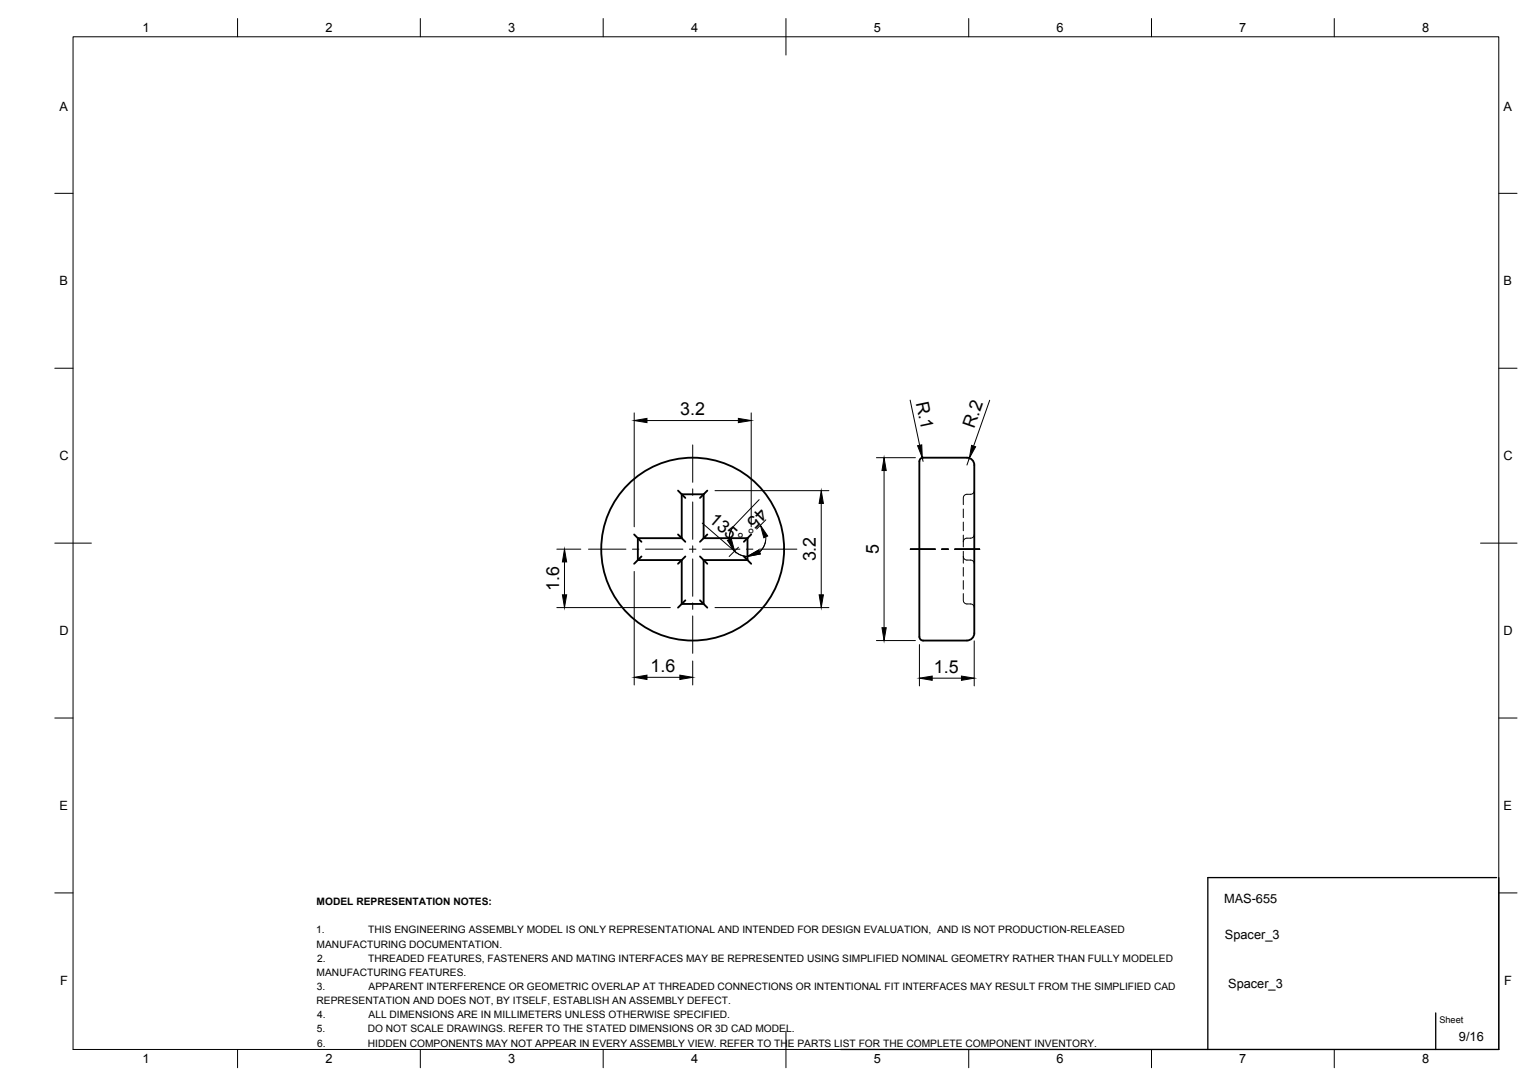
ISO-10303-21;
HEADER;
FILE_DESCRIPTION((''),'2;1');
FILE_NAME('Spacer_3.step','2026-10-09T11:34:15-07:00',(''),(''),'','','');
FILE_SCHEMA (('AUTOMOTIVE_DESIGN { 1 0 10303 214 3 1 1 }'));
ENDSEC;
DATA;
#10=MECHANICAL_DESIGN_GEOMETRIC_PRESENTATION_REPRESENTATION('',(#641),#117170);
#365=ELLIPSE('',#52371,0.141421356237294,0.1) ;
#366=ELLIPSE('',#52372,0.141421356237322,0.1) ;
#367=ELLIPSE('',#52374,0.141421356237325,0.1) ;
#368=ELLIPSE('',#52376,0.141421356237297,0.1) ;
#369=ELLIPSE('',#52378,0.141421356237322,0.1) ;
#370=ELLIPSE('',#52380,0.141421356237297,0.1) ;
#371=ELLIPSE('',#52382,0.141421356237322,0.1) ;
#372=ELLIPSE('',#52384,0.141421356237294,0.1) ;
#373=ELLIPSE('',#52386,0.141421356237325,0.1) ;
#374=ELLIPSE('',#52388,0.141421356237297,0.1) ;
#375=ELLIPSE('',#52390,0.141421356237322,0.1) ;
#376=ELLIPSE('',#52392,0.141421356237297,0.1) ;
#377=ELLIPSE('',#52411,0.141421356237297,0.1) ;
#378=ELLIPSE('',#52412,0.141421356237322,0.1) ;
#379=ELLIPSE('',#52414,0.141421356237322,0.1) ;
#380=ELLIPSE('',#52416,0.141421356237297,0.1) ;
#381=ELLIPSE('',#52418,0.141421356237322,0.1) ;
#382=ELLIPSE('',#52420,0.141421356237297,0.1) ;
#383=ELLIPSE('',#52422,0.141421356237297,0.1) ;
#384=ELLIPSE('',#52423,0.141421356237297,0.1) ;
#385=ELLIPSE('',#52425,0.141421356237322,0.1) ;
#386=ELLIPSE('',#52428,0.141421356237297,0.1) ;
#387=ELLIPSE('',#52430,0.141421356237322,0.1) ;
#388=ELLIPSE('',#52432,0.141421356237297,0.1) ;
#599=SHAPE_REPRESENTATION_RELATIONSHIP('SRR','None',#117254,#620) ;
#620=ADVANCED_BREP_SHAPE_REPRESENTATION('',(#662),#117162) ;
#641=STYLED_ITEM('',(#117355),#662) ;
#662=MANIFOLD_SOLID_BREP('Body1',#49070) ;
#736=FACE_BOUND('',#15495,.T.) ;
#2537=PLANE('',#52394) ;
#2538=PLANE('',#52395) ;
#2539=PLANE('',#52396) ;
#2540=PLANE('',#52397) ;
#2541=PLANE('',#52398) ;
#2542=PLANE('',#52399) ;
#2543=PLANE('',#52400) ;
#2544=PLANE('',#52409) ;
#2545=PLANE('',#52434) ;
#2546=PLANE('',#52435) ;
#2547=PLANE('',#52436) ;
#2548=PLANE('',#52437) ;
#2549=PLANE('',#52441) ;
#2550=PLANE('',#52442) ;
#2551=PLANE('',#52443) ;
#4488=LINE('',#88586,#7702) ;
#4489=LINE('',#88590,#7703) ;
#4490=LINE('',#88594,#7704) ;
#4491=LINE('',#88597,#7705) ;
#4492=LINE('',#88600,#7706) ;
#4493=LINE('',#88603,#7707) ;
#4494=LINE('',#88606,#7708) ;
#4495=LINE('',#88609,#7709) ;
#4496=LINE('',#88612,#7710) ;
#4497=LINE('',#88615,#7711) ;
#4498=LINE('',#88618,#7712) ;
#4499=LINE('',#88620,#7713) ;
#4500=LINE('',#88624,#7714) ;
#4501=LINE('',#88626,#7715) ;
#4502=LINE('',#88630,#7716) ;
#4503=LINE('',#88632,#7717) ;
#4504=LINE('',#88636,#7718) ;
#4505=LINE('',#88638,#7719) ;
#4506=LINE('',#88642,#7720) ;
#4507=LINE('',#88644,#7721) ;
#4508=LINE('',#88648,#7722) ;
#4509=LINE('',#88650,#7723) ;
#4510=LINE('',#88653,#7724) ;
#4511=LINE('',#88654,#7725) ;
#4512=LINE('',#88657,#7726) ;
#4513=LINE('',#88659,#7727) ;
#4514=LINE('',#88660,#7728) ;
#4515=LINE('',#88663,#7729) ;
#4516=LINE('',#88664,#7730) ;
#4517=LINE('',#88667,#7731) ;
#4518=LINE('',#88668,#7732) ;
#4519=LINE('',#88671,#7733) ;
#4520=LINE('',#88672,#7734) ;
#4521=LINE('',#88675,#7735) ;
#4522=LINE('',#88676,#7736) ;
#4523=LINE('',#88679,#7737) ;
#4524=LINE('',#88680,#7738) ;
#4525=LINE('',#88692,#7739) ;
#4526=LINE('',#88700,#7740) ;
#4527=LINE('',#88705,#7741) ;
#4528=LINE('',#88709,#7742) ;
#4529=LINE('',#88713,#7743) ;
#4530=LINE('',#88717,#7744) ;
#4531=LINE('',#88720,#7745) ;
#4532=LINE('',#88724,#7746) ;
#4533=LINE('',#88728,#7747) ;
#4534=LINE('',#88732,#7748) ;
#4535=LINE('',#88734,#7749) ;
#4536=LINE('',#88737,#7750) ;
#4537=LINE('',#88738,#7751) ;
#4538=LINE('',#88741,#7752) ;
#4539=LINE('',#88743,#7753) ;
#4540=LINE('',#88746,#7754) ;
#4541=LINE('',#88748,#7755) ;
#4542=LINE('',#88752,#7756) ;
#4543=LINE('',#88755,#7757) ;
#4544=LINE('',#88757,#7758) ;
#4545=LINE('',#88759,#7759) ;
#4546=LINE('',#88761,#7760) ;
#4547=LINE('',#88768,#7761) ;
#4548=LINE('',#88770,#7762) ;
#7702=VECTOR('',#62675,10.) ;
#7703=VECTOR('',#62678,10.) ;
#7704=VECTOR('',#62683,10.) ;
#7705=VECTOR('',#62686,10.) ;
#7706=VECTOR('',#62689,10.) ;
#7707=VECTOR('',#62692,10.) ;
#7708=VECTOR('',#62695,10.) ;
#7709=VECTOR('',#62698,10.) ;
#7710=VECTOR('',#62701,10.) ;
#7711=VECTOR('',#62704,10.) ;
#7712=VECTOR('',#62707,10.) ;
#7713=VECTOR('',#62708,10.) ;
#7714=VECTOR('',#62713,10.) ;
#7715=VECTOR('',#62714,10.) ;
#7716=VECTOR('',#62719,10.) ;
#7717=VECTOR('',#62720,10.) ;
#7718=VECTOR('',#62725,10.) ;
#7719=VECTOR('',#62726,10.) ;
#7720=VECTOR('',#62731,10.) ;
#7721=VECTOR('',#62732,10.) ;
#7722=VECTOR('',#62737,10.) ;
#7723=VECTOR('',#62738,10.) ;
#7724=VECTOR('',#62743,10.) ;
#7725=VECTOR('',#62744,10.) ;
#7726=VECTOR('',#62747,10.) ;
#7727=VECTOR('',#62748,10.) ;
#7728=VECTOR('',#62749,10.) ;
#7729=VECTOR('',#62752,10.) ;
#7730=VECTOR('',#62753,10.) ;
#7731=VECTOR('',#62756,10.) ;
#7732=VECTOR('',#62757,10.) ;
#7733=VECTOR('',#62760,10.) ;
#7734=VECTOR('',#62761,10.) ;
#7735=VECTOR('',#62764,10.) ;
#7736=VECTOR('',#62765,10.) ;
#7737=VECTOR('',#62768,10.) ;
#7738=VECTOR('',#62769,10.) ;
#7739=VECTOR('',#62784,2.5) ;
#7740=VECTOR('',#62793,10.) ;
#7741=VECTOR('',#62800,10.) ;
#7742=VECTOR('',#62805,10.) ;
#7743=VECTOR('',#62810,10.) ;
#7744=VECTOR('',#62815,10.) ;
#7745=VECTOR('',#62818,10.) ;
#7746=VECTOR('',#62821,10.) ;
#7747=VECTOR('',#62824,10.) ;
#7748=VECTOR('',#62829,10.) ;
#7749=VECTOR('',#62830,10.) ;
#7750=VECTOR('',#62835,10.) ;
#7751=VECTOR('',#62836,10.) ;
#7752=VECTOR('',#62839,10.) ;
#7753=VECTOR('',#62840,10.) ;
#7754=VECTOR('',#62845,10.) ;
#7755=VECTOR('',#62846,10.) ;
#7756=VECTOR('',#62851,10.) ;
#7757=VECTOR('',#62856,10.) ;
#7758=VECTOR('',#62859,10.) ;
#7759=VECTOR('',#62862,10.) ;
#7760=VECTOR('',#62865,10.) ;
#7761=VECTOR('',#62876,10.) ;
#7762=VECTOR('',#62879,10.) ;
#10090=CYLINDRICAL_SURFACE('',#52370,0.1) ;
#10091=CYLINDRICAL_SURFACE('',#52373,0.1) ;
#10092=CYLINDRICAL_SURFACE('',#52375,0.1) ;
#10093=CYLINDRICAL_SURFACE('',#52377,0.1) ;
#10094=CYLINDRICAL_SURFACE('',#52379,0.1) ;
#10095=CYLINDRICAL_SURFACE('',#52381,0.1) ;
#10096=CYLINDRICAL_SURFACE('',#52383,0.1) ;
#10097=CYLINDRICAL_SURFACE('',#52385,0.1) ;
#10098=CYLINDRICAL_SURFACE('',#52387,0.1) ;
#10099=CYLINDRICAL_SURFACE('',#52389,0.1) ;
#10100=CYLINDRICAL_SURFACE('',#52391,0.1) ;
#10101=CYLINDRICAL_SURFACE('',#52393,0.1) ;
#10102=CYLINDRICAL_SURFACE('',#52406,2.5) ;
#10103=CYLINDRICAL_SURFACE('',#52410,0.1) ;
#10104=CYLINDRICAL_SURFACE('',#52413,0.1) ;
#10105=CYLINDRICAL_SURFACE('',#52415,0.1) ;
#10106=CYLINDRICAL_SURFACE('',#52417,0.1) ;
#10107=CYLINDRICAL_SURFACE('',#52419,0.1) ;
#10108=CYLINDRICAL_SURFACE('',#52421,0.1) ;
#10109=CYLINDRICAL_SURFACE('',#52424,0.1) ;
#10110=CYLINDRICAL_SURFACE('',#52426,0.1) ;
#10111=CYLINDRICAL_SURFACE('',#52427,0.1) ;
#10112=CYLINDRICAL_SURFACE('',#52429,0.1) ;
#10113=CYLINDRICAL_SURFACE('',#52431,0.1) ;
#10114=CYLINDRICAL_SURFACE('',#52433,0.1) ;
#12299=FACE_OUTER_BOUND('',#15457,.T.) ;
#12300=FACE_OUTER_BOUND('',#15458,.T.) ;
#12301=FACE_OUTER_BOUND('',#15459,.T.) ;
#12302=FACE_OUTER_BOUND('',#15460,.T.) ;
#12303=FACE_OUTER_BOUND('',#15461,.T.) ;
#12304=FACE_OUTER_BOUND('',#15462,.T.) ;
#12305=FACE_OUTER_BOUND('',#15463,.T.) ;
#12306=FACE_OUTER_BOUND('',#15464,.T.) ;
#12307=FACE_OUTER_BOUND('',#15465,.T.) ;
#12308=FACE_OUTER_BOUND('',#15466,.T.) ;
#12309=FACE_OUTER_BOUND('',#15467,.T.) ;
#12310=FACE_OUTER_BOUND('',#15468,.T.) ;
#12311=FACE_OUTER_BOUND('',#15469,.T.) ;
#12312=FACE_OUTER_BOUND('',#15470,.T.) ;
#12313=FACE_OUTER_BOUND('',#15471,.T.) ;
#12314=FACE_OUTER_BOUND('',#15472,.T.) ;
#12315=FACE_OUTER_BOUND('',#15473,.T.) ;
#12316=FACE_OUTER_BOUND('',#15474,.T.) ;
#12317=FACE_OUTER_BOUND('',#15475,.T.) ;
#12318=FACE_OUTER_BOUND('',#15476,.T.) ;
#12319=FACE_OUTER_BOUND('',#15477,.T.) ;
#12320=FACE_OUTER_BOUND('',#15478,.T.) ;
#12321=FACE_OUTER_BOUND('',#15479,.T.) ;
#12322=FACE_OUTER_BOUND('',#15480,.T.) ;
#12323=FACE_OUTER_BOUND('',#15481,.T.) ;
#12324=FACE_OUTER_BOUND('',#15482,.T.) ;
#12325=FACE_OUTER_BOUND('',#15483,.T.) ;
#12326=FACE_OUTER_BOUND('',#15484,.T.) ;
#12327=FACE_OUTER_BOUND('',#15485,.T.) ;
#12328=FACE_OUTER_BOUND('',#15486,.T.) ;
#12329=FACE_OUTER_BOUND('',#15487,.T.) ;
#12330=FACE_OUTER_BOUND('',#15488,.T.) ;
#12331=FACE_OUTER_BOUND('',#15489,.T.) ;
#12332=FACE_OUTER_BOUND('',#15490,.T.) ;
#12333=FACE_OUTER_BOUND('',#15491,.T.) ;
#12334=FACE_OUTER_BOUND('',#15492,.T.) ;
#12335=FACE_OUTER_BOUND('',#15493,.T.) ;
#12336=FACE_OUTER_BOUND('',#15494,.T.) ;
#12337=FACE_OUTER_BOUND('',#15496,.T.) ;
#12338=FACE_OUTER_BOUND('',#15497,.T.) ;
#12339=FACE_OUTER_BOUND('',#15498,.T.) ;
#12340=FACE_OUTER_BOUND('',#15499,.T.) ;
#15457=EDGE_LOOP('',(#38114,#38115,#38116,#38117)) ;
#15458=EDGE_LOOP('',(#38118,#38119,#38120,#38121)) ;
#15459=EDGE_LOOP('',(#38122,#38123,#38124,#38125)) ;
#15460=EDGE_LOOP('',(#38126,#38127,#38128,#38129)) ;
#15461=EDGE_LOOP('',(#38130,#38131,#38132,#38133)) ;
#15462=EDGE_LOOP('',(#38134,#38135,#38136,#38137)) ;
#15463=EDGE_LOOP('',(#38138,#38139,#38140,#38141)) ;
#15464=EDGE_LOOP('',(#38142,#38143,#38144,#38145)) ;
#15465=EDGE_LOOP('',(#38146,#38147,#38148,#38149)) ;
#15466=EDGE_LOOP('',(#38150,#38151,#38152,#38153)) ;
#15467=EDGE_LOOP('',(#38154,#38155,#38156,#38157)) ;
#15468=EDGE_LOOP('',(#38158,#38159,#38160,#38161)) ;
#15469=EDGE_LOOP('',(#38162,#38163,#38164,#38165)) ;
#15470=EDGE_LOOP('',(#38166,#38167,#38168,#38169)) ;
#15471=EDGE_LOOP('',(#38170,#38171,#38172,#38173)) ;
#15472=EDGE_LOOP('',(#38174,#38175,#38176,#38177)) ;
#15473=EDGE_LOOP('',(#38178,#38179,#38180,#38181)) ;
#15474=EDGE_LOOP('',(#38182,#38183,#38184,#38185)) ;
#15475=EDGE_LOOP('',(#38186,#38187,#38188,#38189,#38190,#38191,#38192,#38193,
#38194,#38195,#38196,#38197)) ;
#15476=EDGE_LOOP('',(#38198,#38199,#38200,#38201,#38202)) ;
#15477=EDGE_LOOP('',(#38203,#38204,#38205,#38206,#38207,#38208)) ;
#15478=EDGE_LOOP('',(#38209)) ;
#15479=EDGE_LOOP('',(#38210,#38211,#38212,#38213)) ;
#15480=EDGE_LOOP('',(#38214,#38215,#38216,#38217)) ;
#15481=EDGE_LOOP('',(#38218,#38219,#38220,#38221)) ;
#15482=EDGE_LOOP('',(#38222,#38223,#38224,#38225)) ;
#15483=EDGE_LOOP('',(#38226,#38227,#38228,#38229)) ;
#15484=EDGE_LOOP('',(#38230,#38231,#38232,#38233)) ;
#15485=EDGE_LOOP('',(#38234,#38235,#38236,#38237)) ;
#15486=EDGE_LOOP('',(#38238,#38239,#38240,#38241)) ;
#15487=EDGE_LOOP('',(#38242,#38243,#38244,#38245)) ;
#15488=EDGE_LOOP('',(#38246,#38247,#38248,#38249)) ;
#15489=EDGE_LOOP('',(#38250,#38251,#38252,#38253)) ;
#15490=EDGE_LOOP('',(#38254,#38255,#38256,#38257)) ;
#15491=EDGE_LOOP('',(#38258,#38259,#38260,#38261)) ;
#15492=EDGE_LOOP('',(#38262,#38263,#38264,#38265)) ;
#15493=EDGE_LOOP('',(#38266,#38267,#38268,#38269)) ;
#15494=EDGE_LOOP('',(#38270)) ;
#15495=EDGE_LOOP('',(#38271,#38272,#38273,#38274,#38275,#38276,#38277,#38278,
#38279,#38280,#38281,#38282)) ;
#15496=EDGE_LOOP('',(#38283,#38284,#38285,#38286,#38287)) ;
#15497=EDGE_LOOP('',(#38288,#38289,#38290,#38291)) ;
#15498=EDGE_LOOP('',(#38292,#38293,#38294,#38295)) ;
#15499=EDGE_LOOP('',(#38296,#38297,#38298,#38299)) ;
#18501=CIRCLE('',#52402,2.4) ;
#18502=CIRCLE('',#52403,0.1) ;
#18503=CIRCLE('',#52404,2.5) ;
#18504=CIRCLE('',#52405,2.5) ;
#18505=CIRCLE('',#52407,2.5) ;
#18506=CIRCLE('',#52408,2.5) ;
#18507=CIRCLE('',#52438,2.3) ;
#18508=CIRCLE('',#52440,0.2) ;
#21615=VERTEX_POINT('',#88584) ;
#21616=VERTEX_POINT('',#88585) ;
#21617=VERTEX_POINT('',#88587) ;
#21618=VERTEX_POINT('',#88589) ;
#21619=VERTEX_POINT('',#88593) ;
#21620=VERTEX_POINT('',#88595) ;
#21621=VERTEX_POINT('',#88599) ;
#21622=VERTEX_POINT('',#88601) ;
#21623=VERTEX_POINT('',#88605) ;
#21624=VERTEX_POINT('',#88607) ;
#21625=VERTEX_POINT('',#88611) ;
#21626=VERTEX_POINT('',#88613) ;
#21627=VERTEX_POINT('',#88617) ;
#21628=VERTEX_POINT('',#88619) ;
#21629=VERTEX_POINT('',#88623) ;
#21630=VERTEX_POINT('',#88625) ;
#21631=VERTEX_POINT('',#88629) ;
#21632=VERTEX_POINT('',#88631) ;
#21633=VERTEX_POINT('',#88635) ;
#21634=VERTEX_POINT('',#88637) ;
#21635=VERTEX_POINT('',#88641) ;
#21636=VERTEX_POINT('',#88643) ;
#21637=VERTEX_POINT('',#88647) ;
#21638=VERTEX_POINT('',#88649) ;
#21639=VERTEX_POINT('',#88656) ;
#21640=VERTEX_POINT('',#88658) ;
#21641=VERTEX_POINT('',#88662) ;
#21642=VERTEX_POINT('',#88666) ;
#21643=VERTEX_POINT('',#88670) ;
#21644=VERTEX_POINT('',#88674) ;
#21645=VERTEX_POINT('',#88678) ;
#21646=VERTEX_POINT('',#88683) ;
#21647=VERTEX_POINT('',#88685) ;
#21648=VERTEX_POINT('',#88687) ;
#21649=VERTEX_POINT('',#88691) ;
#21650=VERTEX_POINT('',#88693) ;
#21651=VERTEX_POINT('',#88698) ;
#21652=VERTEX_POINT('',#88699) ;
#21653=VERTEX_POINT('',#88704) ;
#21654=VERTEX_POINT('',#88708) ;
#21655=VERTEX_POINT('',#88712) ;
#21656=VERTEX_POINT('',#88716) ;
#21657=VERTEX_POINT('',#88718) ;
#21658=VERTEX_POINT('',#88722) ;
#21659=VERTEX_POINT('',#88723) ;
#21660=VERTEX_POINT('',#88725) ;
#21661=VERTEX_POINT('',#88727) ;
#21662=VERTEX_POINT('',#88731) ;
#21663=VERTEX_POINT('',#88733) ;
#21664=VERTEX_POINT('',#88740) ;
#21665=VERTEX_POINT('',#88742) ;
#21666=VERTEX_POINT('',#88747) ;
#21667=VERTEX_POINT('',#88751) ;
#21668=VERTEX_POINT('',#88763) ;
#27335=EDGE_CURVE('',#21615,#21616,#4488,.T.) ;
#27336=EDGE_CURVE('',#21616,#21617,#365,.T.) ;
#27337=EDGE_CURVE('',#21617,#21618,#4489,.T.) ;
#27338=EDGE_CURVE('',#21615,#21618,#366,.T.) ;
#27339=EDGE_CURVE('',#21616,#21619,#4490,.T.) ;
#27340=EDGE_CURVE('',#21619,#21620,#367,.T.) ;
#27341=EDGE_CURVE('',#21620,#21617,#4491,.T.) ;
#27342=EDGE_CURVE('',#21619,#21621,#4492,.T.) ;
#27343=EDGE_CURVE('',#21621,#21622,#368,.T.) ;
#27344=EDGE_CURVE('',#21622,#21620,#4493,.T.) ;
#27345=EDGE_CURVE('',#21621,#21623,#4494,.T.) ;
#27346=EDGE_CURVE('',#21623,#21624,#369,.T.) ;
#27347=EDGE_CURVE('',#21624,#21622,#4495,.T.) ;
#27348=EDGE_CURVE('',#21623,#21625,#4496,.T.) ;
#27349=EDGE_CURVE('',#21625,#21626,#370,.T.) ;
#27350=EDGE_CURVE('',#21626,#21624,#4497,.T.) ;
#27351=EDGE_CURVE('',#21627,#21626,#4498,.T.) ;
#27352=EDGE_CURVE('',#21625,#21628,#4499,.T.) ;
#27353=EDGE_CURVE('',#21628,#21627,#371,.T.) ;
#27354=EDGE_CURVE('',#21629,#21627,#4500,.T.) ;
#27355=EDGE_CURVE('',#21628,#21630,#4501,.T.) ;
#27356=EDGE_CURVE('',#21630,#21629,#372,.T.) ;
#27357=EDGE_CURVE('',#21631,#21629,#4502,.T.) ;
#27358=EDGE_CURVE('',#21630,#21632,#4503,.T.) ;
#27359=EDGE_CURVE('',#21632,#21631,#373,.T.) ;
#27360=EDGE_CURVE('',#21633,#21631,#4504,.T.) ;
#27361=EDGE_CURVE('',#21632,#21634,#4505,.T.) ;
#27362=EDGE_CURVE('',#21634,#21633,#374,.T.) ;
#27363=EDGE_CURVE('',#21635,#21633,#4506,.T.) ;
#27364=EDGE_CURVE('',#21634,#21636,#4507,.T.) ;
#27365=EDGE_CURVE('',#21636,#21635,#375,.T.) ;
#27366=EDGE_CURVE('',#21637,#21635,#4508,.T.) ;
#27367=EDGE_CURVE('',#21636,#21638,#4509,.T.) ;
#27368=EDGE_CURVE('',#21638,#21637,#376,.T.) ;
#27369=EDGE_CURVE('',#21618,#21637,#4510,.T.) ;
#27370=EDGE_CURVE('',#21638,#21615,#4511,.T.) ;
#27371=EDGE_CURVE('',#21639,#21631,#4512,.T.) ;
#27372=EDGE_CURVE('',#21640,#21639,#4513,.T.) ;
#27373=EDGE_CURVE('',#21640,#21629,#4514,.T.) ;
#27374=EDGE_CURVE('',#21641,#21633,#4515,.T.) ;
#27375=EDGE_CURVE('',#21639,#21641,#4516,.T.) ;
#27376=EDGE_CURVE('',#21642,#21635,#4517,.T.) ;
#27377=EDGE_CURVE('',#21641,#21642,#4518,.T.) ;
#27378=EDGE_CURVE('',#21643,#21637,#4519,.T.) ;
#27379=EDGE_CURVE('',#21642,#21643,#4520,.T.) ;
#27380=EDGE_CURVE('',#21644,#21618,#4521,.T.) ;
#27381=EDGE_CURVE('',#21643,#21644,#4522,.T.) ;
#27382=EDGE_CURVE('',#21645,#21617,#4523,.T.) ;
#27383=EDGE_CURVE('',#21644,#21645,#4524,.T.) ;
#27384=EDGE_CURVE('',#21646,#21646,#18501,.T.) ;
#27385=EDGE_CURVE('',#21646,#21647,#18502,.T.) ;
#27386=EDGE_CURVE('',#21647,#21648,#18503,.T.) ;
#27387=EDGE_CURVE('',#21648,#21647,#18504,.T.) ;
#27388=EDGE_CURVE('',#21648,#21649,#4525,.T.) ;
#27389=EDGE_CURVE('',#21650,#21649,#18505,.T.) ;
#27390=EDGE_CURVE('',#21649,#21650,#18506,.T.) ;
#27391=EDGE_CURVE('',#21651,#21652,#4526,.T.) ;
#27392=EDGE_CURVE('',#21652,#21642,#377,.T.) ;
#27393=EDGE_CURVE('',#21651,#21643,#378,.T.) ;
#27394=EDGE_CURVE('',#21652,#21653,#4527,.T.) ;
#27395=EDGE_CURVE('',#21653,#21641,#379,.T.) ;
#27396=EDGE_CURVE('',#21653,#21654,#4528,.T.) ;
#27397=EDGE_CURVE('',#21654,#21639,#380,.T.) ;
#27398=EDGE_CURVE('',#21654,#21655,#4529,.T.) ;
#27399=EDGE_CURVE('',#21655,#21640,#381,.T.) ;
#27400=EDGE_CURVE('',#21655,#21656,#4530,.T.) ;
#27401=EDGE_CURVE('',#21656,#21657,#382,.T.) ;
#27402=EDGE_CURVE('',#21657,#21640,#4531,.T.) ;
#27403=EDGE_CURVE('',#21658,#21659,#4532,.T.) ;
#27404=EDGE_CURVE('',#21659,#21660,#383,.T.) ;
#27405=EDGE_CURVE('',#21660,#21661,#4533,.T.) ;
#27406=EDGE_CURVE('',#21661,#21658,#384,.T.) ;
#27407=EDGE_CURVE('',#21662,#21660,#4534,.T.) ;
#27408=EDGE_CURVE('',#21659,#21663,#4535,.T.) ;
#27409=EDGE_CURVE('',#21663,#21662,#385,.T.) ;
#27410=EDGE_CURVE('',#21656,#21658,#4536,.T.) ;
#27411=EDGE_CURVE('',#21661,#21657,#4537,.T.) ;
#27412=EDGE_CURVE('',#21664,#21662,#4538,.T.) ;
#27413=EDGE_CURVE('',#21663,#21665,#4539,.T.) ;
#27414=EDGE_CURVE('',#21665,#21664,#386,.T.) ;
#27415=EDGE_CURVE('',#21645,#21664,#4540,.T.) ;
#27416=EDGE_CURVE('',#21665,#21666,#4541,.T.) ;
#27417=EDGE_CURVE('',#21666,#21645,#387,.T.) ;
#27418=EDGE_CURVE('',#21666,#21667,#4542,.T.) ;
#27419=EDGE_CURVE('',#21667,#21644,#388,.T.) ;
#27420=EDGE_CURVE('',#21667,#21651,#4543,.T.) ;
#27421=EDGE_CURVE('',#21657,#21627,#4544,.T.) ;
#27422=EDGE_CURVE('',#21661,#21626,#4545,.T.) ;
#27423=EDGE_CURVE('',#21660,#21624,#4546,.T.) ;
#27424=EDGE_CURVE('',#21668,#21668,#18507,.T.) ;
#27425=EDGE_CURVE('',#21650,#21668,#18508,.T.) ;
#27426=EDGE_CURVE('',#21664,#21620,#4547,.T.) ;
#27427=EDGE_CURVE('',#21662,#21622,#4548,.T.) ;
#38114=ORIENTED_EDGE('',*,*,#27335,.T.) ;
#38115=ORIENTED_EDGE('',*,*,#27336,.T.) ;
#38116=ORIENTED_EDGE('',*,*,#27337,.T.) ;
#38117=ORIENTED_EDGE('',*,*,#27338,.F.) ;
#38118=ORIENTED_EDGE('',*,*,#27339,.T.) ;
#38119=ORIENTED_EDGE('',*,*,#27340,.T.) ;
#38120=ORIENTED_EDGE('',*,*,#27341,.T.) ;
#38121=ORIENTED_EDGE('',*,*,#27336,.F.) ;
#38122=ORIENTED_EDGE('',*,*,#27342,.T.) ;
#38123=ORIENTED_EDGE('',*,*,#27343,.T.) ;
#38124=ORIENTED_EDGE('',*,*,#27344,.T.) ;
#38125=ORIENTED_EDGE('',*,*,#27340,.F.) ;
#38126=ORIENTED_EDGE('',*,*,#27345,.T.) ;
#38127=ORIENTED_EDGE('',*,*,#27346,.T.) ;
#38128=ORIENTED_EDGE('',*,*,#27347,.T.) ;
#38129=ORIENTED_EDGE('',*,*,#27343,.F.) ;
#38130=ORIENTED_EDGE('',*,*,#27348,.T.) ;
#38131=ORIENTED_EDGE('',*,*,#27349,.T.) ;
#38132=ORIENTED_EDGE('',*,*,#27350,.T.) ;
#38133=ORIENTED_EDGE('',*,*,#27346,.F.) ;
#38134=ORIENTED_EDGE('',*,*,#27351,.T.) ;
#38135=ORIENTED_EDGE('',*,*,#27349,.F.) ;
#38136=ORIENTED_EDGE('',*,*,#27352,.T.) ;
#38137=ORIENTED_EDGE('',*,*,#27353,.T.) ;
#38138=ORIENTED_EDGE('',*,*,#27354,.T.) ;
#38139=ORIENTED_EDGE('',*,*,#27353,.F.) ;
#38140=ORIENTED_EDGE('',*,*,#27355,.T.) ;
#38141=ORIENTED_EDGE('',*,*,#27356,.T.) ;
#38142=ORIENTED_EDGE('',*,*,#27357,.T.) ;
#38143=ORIENTED_EDGE('',*,*,#27356,.F.) ;
#38144=ORIENTED_EDGE('',*,*,#27358,.T.) ;
#38145=ORIENTED_EDGE('',*,*,#27359,.T.) ;
#38146=ORIENTED_EDGE('',*,*,#27360,.T.) ;
#38147=ORIENTED_EDGE('',*,*,#27359,.F.) ;
#38148=ORIENTED_EDGE('',*,*,#27361,.T.) ;
#38149=ORIENTED_EDGE('',*,*,#27362,.T.) ;
#38150=ORIENTED_EDGE('',*,*,#27363,.T.) ;
#38151=ORIENTED_EDGE('',*,*,#27362,.F.) ;
#38152=ORIENTED_EDGE('',*,*,#27364,.T.) ;
#38153=ORIENTED_EDGE('',*,*,#27365,.T.) ;
#38154=ORIENTED_EDGE('',*,*,#27366,.T.) ;
#38155=ORIENTED_EDGE('',*,*,#27365,.F.) ;
#38156=ORIENTED_EDGE('',*,*,#27367,.T.) ;
#38157=ORIENTED_EDGE('',*,*,#27368,.T.) ;
#38158=ORIENTED_EDGE('',*,*,#27369,.T.) ;
#38159=ORIENTED_EDGE('',*,*,#27368,.F.) ;
#38160=ORIENTED_EDGE('',*,*,#27370,.T.) ;
#38161=ORIENTED_EDGE('',*,*,#27338,.T.) ;
#38162=ORIENTED_EDGE('',*,*,#27357,.F.) ;
#38163=ORIENTED_EDGE('',*,*,#27371,.F.) ;
#38164=ORIENTED_EDGE('',*,*,#27372,.F.) ;
#38165=ORIENTED_EDGE('',*,*,#27373,.T.) ;
#38166=ORIENTED_EDGE('',*,*,#27360,.F.) ;
#38167=ORIENTED_EDGE('',*,*,#27374,.F.) ;
#38168=ORIENTED_EDGE('',*,*,#27375,.F.) ;
#38169=ORIENTED_EDGE('',*,*,#27371,.T.) ;
#38170=ORIENTED_EDGE('',*,*,#27363,.F.) ;
#38171=ORIENTED_EDGE('',*,*,#27376,.F.) ;
#38172=ORIENTED_EDGE('',*,*,#27377,.F.) ;
#38173=ORIENTED_EDGE('',*,*,#27374,.T.) ;
#38174=ORIENTED_EDGE('',*,*,#27366,.F.) ;
#38175=ORIENTED_EDGE('',*,*,#27378,.F.) ;
#38176=ORIENTED_EDGE('',*,*,#27379,.F.) ;
#38177=ORIENTED_EDGE('',*,*,#27376,.T.) ;
#38178=ORIENTED_EDGE('',*,*,#27369,.F.) ;
#38179=ORIENTED_EDGE('',*,*,#27380,.F.) ;
#38180=ORIENTED_EDGE('',*,*,#27381,.F.) ;
#38181=ORIENTED_EDGE('',*,*,#27378,.T.) ;
#38182=ORIENTED_EDGE('',*,*,#27337,.F.) ;
#38183=ORIENTED_EDGE('',*,*,#27382,.F.) ;
#38184=ORIENTED_EDGE('',*,*,#27383,.F.) ;
#38185=ORIENTED_EDGE('',*,*,#27380,.T.) ;
#38186=ORIENTED_EDGE('',*,*,#27335,.F.) ;
#38187=ORIENTED_EDGE('',*,*,#27370,.F.) ;
#38188=ORIENTED_EDGE('',*,*,#27367,.F.) ;
#38189=ORIENTED_EDGE('',*,*,#27364,.F.) ;
#38190=ORIENTED_EDGE('',*,*,#27361,.F.) ;
#38191=ORIENTED_EDGE('',*,*,#27358,.F.) ;
#38192=ORIENTED_EDGE('',*,*,#27355,.F.) ;
#38193=ORIENTED_EDGE('',*,*,#27352,.F.) ;
#38194=ORIENTED_EDGE('',*,*,#27348,.F.) ;
#38195=ORIENTED_EDGE('',*,*,#27345,.F.) ;
#38196=ORIENTED_EDGE('',*,*,#27342,.F.) ;
#38197=ORIENTED_EDGE('',*,*,#27339,.F.) ;
#38198=ORIENTED_EDGE('',*,*,#27384,.T.) ;
#38199=ORIENTED_EDGE('',*,*,#27385,.T.) ;
#38200=ORIENTED_EDGE('',*,*,#27386,.T.) ;
#38201=ORIENTED_EDGE('',*,*,#27387,.T.) ;
#38202=ORIENTED_EDGE('',*,*,#27385,.F.) ;
#38203=ORIENTED_EDGE('',*,*,#27387,.F.) ;
#38204=ORIENTED_EDGE('',*,*,#27388,.T.) ;
#38205=ORIENTED_EDGE('',*,*,#27389,.F.) ;
#38206=ORIENTED_EDGE('',*,*,#27390,.F.) ;
#38207=ORIENTED_EDGE('',*,*,#27388,.F.) ;
#38208=ORIENTED_EDGE('',*,*,#27386,.F.) ;
#38209=ORIENTED_EDGE('',*,*,#27384,.F.) ;
#38210=ORIENTED_EDGE('',*,*,#27391,.T.) ;
#38211=ORIENTED_EDGE('',*,*,#27392,.T.) ;
#38212=ORIENTED_EDGE('',*,*,#27379,.T.) ;
#38213=ORIENTED_EDGE('',*,*,#27393,.F.) ;
#38214=ORIENTED_EDGE('',*,*,#27394,.T.) ;
#38215=ORIENTED_EDGE('',*,*,#27395,.T.) ;
#38216=ORIENTED_EDGE('',*,*,#27377,.T.) ;
#38217=ORIENTED_EDGE('',*,*,#27392,.F.) ;
#38218=ORIENTED_EDGE('',*,*,#27396,.T.) ;
#38219=ORIENTED_EDGE('',*,*,#27397,.T.) ;
#38220=ORIENTED_EDGE('',*,*,#27375,.T.) ;
#38221=ORIENTED_EDGE('',*,*,#27395,.F.) ;
#38222=ORIENTED_EDGE('',*,*,#27398,.T.) ;
#38223=ORIENTED_EDGE('',*,*,#27399,.T.) ;
#38224=ORIENTED_EDGE('',*,*,#27372,.T.) ;
#38225=ORIENTED_EDGE('',*,*,#27397,.F.) ;
#38226=ORIENTED_EDGE('',*,*,#27400,.T.) ;
#38227=ORIENTED_EDGE('',*,*,#27401,.T.) ;
#38228=ORIENTED_EDGE('',*,*,#27402,.T.) ;
#38229=ORIENTED_EDGE('',*,*,#27399,.F.) ;
#38230=ORIENTED_EDGE('',*,*,#27403,.T.) ;
#38231=ORIENTED_EDGE('',*,*,#27404,.T.) ;
#38232=ORIENTED_EDGE('',*,*,#27405,.T.) ;
#38233=ORIENTED_EDGE('',*,*,#27406,.T.) ;
#38234=ORIENTED_EDGE('',*,*,#27407,.T.) ;
#38235=ORIENTED_EDGE('',*,*,#27404,.F.) ;
#38236=ORIENTED_EDGE('',*,*,#27408,.T.) ;
#38237=ORIENTED_EDGE('',*,*,#27409,.T.) ;
#38238=ORIENTED_EDGE('',*,*,#27410,.T.) ;
#38239=ORIENTED_EDGE('',*,*,#27406,.F.) ;
#38240=ORIENTED_EDGE('',*,*,#27411,.T.) ;
#38241=ORIENTED_EDGE('',*,*,#27401,.F.) ;
#38242=ORIENTED_EDGE('',*,*,#27412,.T.) ;
#38243=ORIENTED_EDGE('',*,*,#27409,.F.) ;
#38244=ORIENTED_EDGE('',*,*,#27413,.T.) ;
#38245=ORIENTED_EDGE('',*,*,#27414,.T.) ;
#38246=ORIENTED_EDGE('',*,*,#27415,.T.) ;
#38247=ORIENTED_EDGE('',*,*,#27414,.F.) ;
#38248=ORIENTED_EDGE('',*,*,#27416,.T.) ;
#38249=ORIENTED_EDGE('',*,*,#27417,.T.) ;
#38250=ORIENTED_EDGE('',*,*,#27383,.T.) ;
#38251=ORIENTED_EDGE('',*,*,#27417,.F.) ;
#38252=ORIENTED_EDGE('',*,*,#27418,.T.) ;
#38253=ORIENTED_EDGE('',*,*,#27419,.T.) ;
#38254=ORIENTED_EDGE('',*,*,#27381,.T.) ;
#38255=ORIENTED_EDGE('',*,*,#27419,.F.) ;
#38256=ORIENTED_EDGE('',*,*,#27420,.T.) ;
#38257=ORIENTED_EDGE('',*,*,#27393,.T.) ;
#38258=ORIENTED_EDGE('',*,*,#27354,.F.) ;
#38259=ORIENTED_EDGE('',*,*,#27373,.F.) ;
#38260=ORIENTED_EDGE('',*,*,#27402,.F.) ;
#38261=ORIENTED_EDGE('',*,*,#27421,.T.) ;
#38262=ORIENTED_EDGE('',*,*,#27351,.F.) ;
#38263=ORIENTED_EDGE('',*,*,#27421,.F.) ;
#38264=ORIENTED_EDGE('',*,*,#27411,.F.) ;
#38265=ORIENTED_EDGE('',*,*,#27422,.T.) ;
#38266=ORIENTED_EDGE('',*,*,#27350,.F.) ;
#38267=ORIENTED_EDGE('',*,*,#27422,.F.) ;
#38268=ORIENTED_EDGE('',*,*,#27405,.F.) ;
#38269=ORIENTED_EDGE('',*,*,#27423,.T.) ;
#38270=ORIENTED_EDGE('',*,*,#27424,.F.) ;
#38271=ORIENTED_EDGE('',*,*,#27403,.F.) ;
#38272=ORIENTED_EDGE('',*,*,#27410,.F.) ;
#38273=ORIENTED_EDGE('',*,*,#27400,.F.) ;
#38274=ORIENTED_EDGE('',*,*,#27398,.F.) ;
#38275=ORIENTED_EDGE('',*,*,#27396,.F.) ;
#38276=ORIENTED_EDGE('',*,*,#27394,.F.) ;
#38277=ORIENTED_EDGE('',*,*,#27391,.F.) ;
#38278=ORIENTED_EDGE('',*,*,#27420,.F.) ;
#38279=ORIENTED_EDGE('',*,*,#27418,.F.) ;
#38280=ORIENTED_EDGE('',*,*,#27416,.F.) ;
#38281=ORIENTED_EDGE('',*,*,#27413,.F.) ;
#38282=ORIENTED_EDGE('',*,*,#27408,.F.) ;
#38283=ORIENTED_EDGE('',*,*,#27389,.T.) ;
#38284=ORIENTED_EDGE('',*,*,#27390,.T.) ;
#38285=ORIENTED_EDGE('',*,*,#27425,.T.) ;
#38286=ORIENTED_EDGE('',*,*,#27424,.T.) ;
#38287=ORIENTED_EDGE('',*,*,#27425,.F.) ;
#38288=ORIENTED_EDGE('',*,*,#27341,.F.) ;
#38289=ORIENTED_EDGE('',*,*,#27426,.F.) ;
#38290=ORIENTED_EDGE('',*,*,#27415,.F.) ;
#38291=ORIENTED_EDGE('',*,*,#27382,.T.) ;
#38292=ORIENTED_EDGE('',*,*,#27344,.F.) ;
#38293=ORIENTED_EDGE('',*,*,#27427,.F.) ;
#38294=ORIENTED_EDGE('',*,*,#27412,.F.) ;
#38295=ORIENTED_EDGE('',*,*,#27426,.T.) ;
#38296=ORIENTED_EDGE('',*,*,#27347,.F.) ;
#38297=ORIENTED_EDGE('',*,*,#27423,.F.) ;
#38298=ORIENTED_EDGE('',*,*,#27407,.F.) ;
#38299=ORIENTED_EDGE('',*,*,#27427,.T.) ;
#45711=TOROIDAL_SURFACE('',#52401,2.4,0.1) ;
#45712=TOROIDAL_SURFACE('',#52439,2.3,0.2) ;
#47517=ADVANCED_FACE('',(#12299),#10090,.F.) ;
#47518=ADVANCED_FACE('',(#12300),#10091,.F.) ;
#47519=ADVANCED_FACE('',(#12301),#10092,.F.) ;
#47520=ADVANCED_FACE('',(#12302),#10093,.F.) ;
#47521=ADVANCED_FACE('',(#12303),#10094,.F.) ;
#47522=ADVANCED_FACE('',(#12304),#10095,.F.) ;
#47523=ADVANCED_FACE('',(#12305),#10096,.F.) ;
#47524=ADVANCED_FACE('',(#12306),#10097,.F.) ;
#47525=ADVANCED_FACE('',(#12307),#10098,.F.) ;
#47526=ADVANCED_FACE('',(#12308),#10099,.F.) ;
#47527=ADVANCED_FACE('',(#12309),#10100,.F.) ;
#47528=ADVANCED_FACE('',(#12310),#10101,.F.) ;
#47529=ADVANCED_FACE('',(#12311),#2537,.F.) ;
#47530=ADVANCED_FACE('',(#12312),#2538,.F.) ;
#47531=ADVANCED_FACE('',(#12313),#2539,.F.) ;
#47532=ADVANCED_FACE('',(#12314),#2540,.F.) ;
#47533=ADVANCED_FACE('',(#12315),#2541,.F.) ;
#47534=ADVANCED_FACE('',(#12316),#2542,.F.) ;
#47535=ADVANCED_FACE('',(#12317),#2543,.F.) ;
#47536=ADVANCED_FACE('',(#12318),#45711,.T.) ;
#47537=ADVANCED_FACE('',(#12319),#10102,.T.) ;
#47538=ADVANCED_FACE('',(#12320),#2544,.T.) ;
#47539=ADVANCED_FACE('',(#12321),#10103,.T.) ;
#47540=ADVANCED_FACE('',(#12322),#10104,.T.) ;
#47541=ADVANCED_FACE('',(#12323),#10105,.T.) ;
#47542=ADVANCED_FACE('',(#12324),#10106,.T.) ;
#47543=ADVANCED_FACE('',(#12325),#10107,.T.) ;
#47544=ADVANCED_FACE('',(#12326),#10108,.T.) ;
#47545=ADVANCED_FACE('',(#12327),#10109,.T.) ;
#47546=ADVANCED_FACE('',(#12328),#10110,.T.) ;
#47547=ADVANCED_FACE('',(#12329),#10111,.T.) ;
#47548=ADVANCED_FACE('',(#12330),#10112,.T.) ;
#47549=ADVANCED_FACE('',(#12331),#10113,.T.) ;
#47550=ADVANCED_FACE('',(#12332),#10114,.T.) ;
#47551=ADVANCED_FACE('',(#12333),#2545,.F.) ;
#47552=ADVANCED_FACE('',(#12334),#2546,.F.) ;
#47553=ADVANCED_FACE('',(#12335),#2547,.F.) ;
#47554=ADVANCED_FACE('',(#12336,#736),#2548,.F.) ;
#47555=ADVANCED_FACE('',(#12337),#45712,.T.) ;
#47556=ADVANCED_FACE('',(#12338),#2549,.F.) ;
#47557=ADVANCED_FACE('',(#12339),#2550,.F.) ;
#47558=ADVANCED_FACE('',(#12340),#2551,.F.) ;
#49070=CLOSED_SHELL('',(#47517,#47518,#47519,#47520,#47521,#47522,#47523,
#47524,#47525,#47526,#47527,#47528,#47529,#47530,#47531,#47532,#47533,#47534,
#47535,#47536,#47537,#47538,#47539,#47540,#47541,#47542,#47543,#47544,#47545,
#47546,#47547,#47548,#47549,#47550,#47551,#47552,#47553,#47554,#47555,#47556,
#47557,#47558)) ;
#52369=AXIS2_PLACEMENT_3D('',#88582,#62671,#62672) ;
#52370=AXIS2_PLACEMENT_3D('',#88583,#62673,#62674) ;
#52371=AXIS2_PLACEMENT_3D('',#88588,#62676,#62677) ;
#52372=AXIS2_PLACEMENT_3D('',#88591,#62679,#62680) ;
#52373=AXIS2_PLACEMENT_3D('',#88592,#62681,#62682) ;
#52374=AXIS2_PLACEMENT_3D('',#88596,#62684,#62685) ;
#52375=AXIS2_PLACEMENT_3D('',#88598,#62687,#62688) ;
#52376=AXIS2_PLACEMENT_3D('',#88602,#62690,#62691) ;
#52377=AXIS2_PLACEMENT_3D('',#88604,#62693,#62694) ;
#52378=AXIS2_PLACEMENT_3D('',#88608,#62696,#62697) ;
#52379=AXIS2_PLACEMENT_3D('',#88610,#62699,#62700) ;
#52380=AXIS2_PLACEMENT_3D('',#88614,#62702,#62703) ;
#52381=AXIS2_PLACEMENT_3D('',#88616,#62705,#62706) ;
#52382=AXIS2_PLACEMENT_3D('',#88621,#62709,#62710) ;
#52383=AXIS2_PLACEMENT_3D('',#88622,#62711,#62712) ;
#52384=AXIS2_PLACEMENT_3D('',#88627,#62715,#62716) ;
#52385=AXIS2_PLACEMENT_3D('',#88628,#62717,#62718) ;
#52386=AXIS2_PLACEMENT_3D('',#88633,#62721,#62722) ;
#52387=AXIS2_PLACEMENT_3D('',#88634,#62723,#62724) ;
#52388=AXIS2_PLACEMENT_3D('',#88639,#62727,#62728) ;
#52389=AXIS2_PLACEMENT_3D('',#88640,#62729,#62730) ;
#52390=AXIS2_PLACEMENT_3D('',#88645,#62733,#62734) ;
#52391=AXIS2_PLACEMENT_3D('',#88646,#62735,#62736) ;
#52392=AXIS2_PLACEMENT_3D('',#88651,#62739,#62740) ;
#52393=AXIS2_PLACEMENT_3D('',#88652,#62741,#62742) ;
#52394=AXIS2_PLACEMENT_3D('',#88655,#62745,#62746) ;
#52395=AXIS2_PLACEMENT_3D('',#88661,#62750,#62751) ;
#52396=AXIS2_PLACEMENT_3D('',#88665,#62754,#62755) ;
#52397=AXIS2_PLACEMENT_3D('',#88669,#62758,#62759) ;
#52398=AXIS2_PLACEMENT_3D('',#88673,#62762,#62763) ;
#52399=AXIS2_PLACEMENT_3D('',#88677,#62766,#62767) ;
#52400=AXIS2_PLACEMENT_3D('',#88681,#62770,#62771) ;
#52401=AXIS2_PLACEMENT_3D('',#88682,#62772,#62773) ;
#52402=AXIS2_PLACEMENT_3D('',#88684,#62774,#62775) ;
#52403=AXIS2_PLACEMENT_3D('',#88686,#62776,#62777) ;
#52404=AXIS2_PLACEMENT_3D('',#88688,#62778,#62779) ;
#52405=AXIS2_PLACEMENT_3D('',#88689,#62780,#62781) ;
#52406=AXIS2_PLACEMENT_3D('',#88690,#62782,#62783) ;
#52407=AXIS2_PLACEMENT_3D('',#88694,#62785,#62786) ;
#52408=AXIS2_PLACEMENT_3D('',#88695,#62787,#62788) ;
#52409=AXIS2_PLACEMENT_3D('',#88696,#62789,#62790) ;
#52410=AXIS2_PLACEMENT_3D('',#88697,#62791,#62792) ;
#52411=AXIS2_PLACEMENT_3D('',#88701,#62794,#62795) ;
#52412=AXIS2_PLACEMENT_3D('',#88702,#62796,#62797) ;
#52413=AXIS2_PLACEMENT_3D('',#88703,#62798,#62799) ;
#52414=AXIS2_PLACEMENT_3D('',#88706,#62801,#62802) ;
#52415=AXIS2_PLACEMENT_3D('',#88707,#62803,#62804) ;
#52416=AXIS2_PLACEMENT_3D('',#88710,#62806,#62807) ;
#52417=AXIS2_PLACEMENT_3D('',#88711,#62808,#62809) ;
#52418=AXIS2_PLACEMENT_3D('',#88714,#62811,#62812) ;
#52419=AXIS2_PLACEMENT_3D('',#88715,#62813,#62814) ;
#52420=AXIS2_PLACEMENT_3D('',#88719,#62816,#62817) ;
#52421=AXIS2_PLACEMENT_3D('',#88721,#62819,#62820) ;
#52422=AXIS2_PLACEMENT_3D('',#88726,#62822,#62823) ;
#52423=AXIS2_PLACEMENT_3D('',#88729,#62825,#62826) ;
#52424=AXIS2_PLACEMENT_3D('',#88730,#62827,#62828) ;
#52425=AXIS2_PLACEMENT_3D('',#88735,#62831,#62832) ;
#52426=AXIS2_PLACEMENT_3D('',#88736,#62833,#62834) ;
#52427=AXIS2_PLACEMENT_3D('',#88739,#62837,#62838) ;
#52428=AXIS2_PLACEMENT_3D('',#88744,#62841,#62842) ;
#52429=AXIS2_PLACEMENT_3D('',#88745,#62843,#62844) ;
#52430=AXIS2_PLACEMENT_3D('',#88749,#62847,#62848) ;
#52431=AXIS2_PLACEMENT_3D('',#88750,#62849,#62850) ;
#52432=AXIS2_PLACEMENT_3D('',#88753,#62852,#62853) ;
#52433=AXIS2_PLACEMENT_3D('',#88754,#62854,#62855) ;
#52434=AXIS2_PLACEMENT_3D('',#88756,#62857,#62858) ;
#52435=AXIS2_PLACEMENT_3D('',#88758,#62860,#62861) ;
#52436=AXIS2_PLACEMENT_3D('',#88760,#62863,#62864) ;
#52437=AXIS2_PLACEMENT_3D('',#88762,#62866,#62867) ;
#52438=AXIS2_PLACEMENT_3D('',#88764,#62868,#62869) ;
#52439=AXIS2_PLACEMENT_3D('',#88765,#62870,#62871) ;
#52440=AXIS2_PLACEMENT_3D('',#88766,#62872,#62873) ;
#52441=AXIS2_PLACEMENT_3D('',#88767,#62874,#62875) ;
#52442=AXIS2_PLACEMENT_3D('',#88769,#62877,#62878) ;
#52443=AXIS2_PLACEMENT_3D('',#88771,#62880,#62881) ;
#62671=DIRECTION('axis',(0.,0.,1.)) ;
#62672=DIRECTION('refdir',(1.,0.,0.)) ;
#62673=DIRECTION('center_axis',(-1.,0.,0.)) ;
#62674=DIRECTION('ref_axis',(0.,-0.707106781186485,-0.70710678118661)) ;
#62675=DIRECTION('',(-1.,0.,0.)) ;
#62676=DIRECTION('center_axis',(-0.707106781186626,0.707106781186469,0.)) ;
#62677=DIRECTION('ref_axis',(0.707106781186469,0.707106781186626,0.)) ;
#62678=DIRECTION('',(1.,0.,0.)) ;
#62679=DIRECTION('center_axis',(-0.70710678118661,0.707106781186485,0.)) ;
#62680=DIRECTION('ref_axis',(-0.707106781186485,-0.70710678118661,0.)) ;
#62681=DIRECTION('center_axis',(-1.41426179436738E-51,1.,0.)) ;
#62682=DIRECTION('ref_axis',(-0.707106781186548,-1.00003410517023E-51,-0.707106781186548)) ;
#62683=DIRECTION('',(-1.41426179436738E-51,1.,0.)) ;
#62684=DIRECTION('center_axis',(0.707106781186626,0.707106781186469,0.)) ;
#62685=DIRECTION('ref_axis',(0.707106781186469,-0.707106781186626,0.)) ;
#62686=DIRECTION('',(1.41426179436738E-51,-1.,0.)) ;
#62687=DIRECTION('center_axis',(1.,0.,0.)) ;
#62688=DIRECTION('ref_axis',(0.,0.707106781186485,-0.70710678118661)) ;
#62689=DIRECTION('',(1.,0.,0.)) ;
#62690=DIRECTION('center_axis',(0.70710678118661,0.707106781186485,0.)) ;
#62691=DIRECTION('ref_axis',(-0.707106781186485,0.70710678118661,0.)) ;
#62692=DIRECTION('',(-1.,0.,0.)) ;
#62693=DIRECTION('center_axis',(-1.41426179436738E-51,1.,0.)) ;
#62694=DIRECTION('ref_axis',(-0.707106781186548,-1.00003410517023E-51,-0.707106781186548)) ;
#62695=DIRECTION('',(-1.41426179436738E-51,1.,0.)) ;
#62696=DIRECTION('center_axis',(0.70710678118661,0.707106781186485,0.)) ;
#62697=DIRECTION('ref_axis',(0.707106781186485,-0.70710678118661,0.)) ;
#62698=DIRECTION('',(1.41426179436738E-51,-1.,0.)) ;
#62699=DIRECTION('center_axis',(1.,0.,0.)) ;
#62700=DIRECTION('ref_axis',(0.,0.707106781186485,-0.70710678118661)) ;
#62701=DIRECTION('',(1.,0.,0.)) ;
#62702=DIRECTION('center_axis',(0.70710678118661,-0.707106781186485,0.)) ;
#62703=DIRECTION('ref_axis',(-0.707106781186485,-0.70710678118661,0.)) ;
#62704=DIRECTION('',(-1.,0.,0.)) ;
#62705=DIRECTION('center_axis',(1.41426179436738E-51,-1.,0.)) ;
#62706=DIRECTION('ref_axis',(0.707106781186548,1.00003410517023E-51,-0.707106781186548)) ;
#62707=DIRECTION('',(-1.41426179436738E-51,1.,0.)) ;
#62708=DIRECTION('',(1.41426179436738E-51,-1.,0.)) ;
#62709=DIRECTION('center_axis',(0.70710678118661,-0.707106781186485,0.)) ;
#62710=DIRECTION('ref_axis',(0.707106781186485,0.70710678118661,0.)) ;
#62711=DIRECTION('center_axis',(1.,0.,0.)) ;
#62712=DIRECTION('ref_axis',(0.,0.707106781186485,-0.70710678118661)) ;
#62713=DIRECTION('',(-1.,0.,0.)) ;
#62714=DIRECTION('',(1.,0.,0.)) ;
#62715=DIRECTION('center_axis',(0.707106781186626,-0.707106781186469,0.)) ;
#62716=DIRECTION('ref_axis',(-0.707106781186469,-0.707106781186626,0.)) ;
#62717=DIRECTION('center_axis',(1.41426179436738E-51,-1.,0.)) ;
#62718=DIRECTION('ref_axis',(0.707106781186548,1.00003410517023E-51,-0.707106781186548)) ;
#62719=DIRECTION('',(-1.41426179436738E-51,1.,0.)) ;
#62720=DIRECTION('',(1.41426179436738E-51,-1.,0.)) ;
#62721=DIRECTION('center_axis',(-0.707106781186626,-0.707106781186469,0.)) ;
#62722=DIRECTION('ref_axis',(-0.707106781186469,0.707106781186626,0.)) ;
#62723=DIRECTION('center_axis',(-1.,0.,0.)) ;
#62724=DIRECTION('ref_axis',(0.,-0.707106781186485,-0.70710678118661)) ;
#62725=DIRECTION('',(1.,0.,0.)) ;
#62726=DIRECTION('',(-1.,0.,0.)) ;
#62727=DIRECTION('center_axis',(-0.70710678118661,-0.707106781186485,0.)) ;
#62728=DIRECTION('ref_axis',(0.707106781186485,-0.70710678118661,0.)) ;
#62729=DIRECTION('center_axis',(1.41426179436738E-51,-1.,0.)) ;
#62730=DIRECTION('ref_axis',(0.707106781186548,1.00003410517023E-51,-0.707106781186548)) ;
#62731=DIRECTION('',(-1.41426179436738E-51,1.,0.)) ;
#62732=DIRECTION('',(1.41426179436738E-51,-1.,0.)) ;
#62733=DIRECTION('center_axis',(-0.70710678118661,-0.707106781186485,0.)) ;
#62734=DIRECTION('ref_axis',(-0.707106781186485,0.70710678118661,0.)) ;
#62735=DIRECTION('center_axis',(-1.,0.,0.)) ;
#62736=DIRECTION('ref_axis',(0.,-0.707106781186485,-0.70710678118661)) ;
#62737=DIRECTION('',(1.,0.,0.)) ;
#62738=DIRECTION('',(-1.,0.,0.)) ;
#62739=DIRECTION('center_axis',(-0.70710678118661,0.707106781186485,0.)) ;
#62740=DIRECTION('ref_axis',(0.707106781186485,0.70710678118661,0.)) ;
#62741=DIRECTION('center_axis',(-1.41426179436738E-51,1.,0.)) ;
#62742=DIRECTION('ref_axis',(-0.707106781186548,-1.00003410517023E-51,-0.707106781186548)) ;
#62743=DIRECTION('',(1.41426179436738E-51,-1.,0.)) ;
#62744=DIRECTION('',(-1.41426179436738E-51,1.,0.)) ;
#62745=DIRECTION('center_axis',(1.,1.41426179436738E-51,0.)) ;
#62746=DIRECTION('ref_axis',(1.41426179436738E-51,-1.,-5.60383084497445E-34)) ;
#62747=DIRECTION('',(0.,0.,-1.)) ;
#62748=DIRECTION('',(1.41426179436738E-51,-1.,-5.60383084497445E-34)) ;
#62749=DIRECTION('',(0.,0.,-1.)) ;
#62750=DIRECTION('center_axis',(0.,-1.,0.)) ;
#62751=DIRECTION('ref_axis',(-1.,0.,-2.52374105052742E-18)) ;
#62752=DIRECTION('',(0.,0.,-1.)) ;
#62753=DIRECTION('',(-1.,0.,-2.52374105052742E-18)) ;
#62754=DIRECTION('center_axis',(1.,1.41426179436738E-51,0.)) ;
#62755=DIRECTION('ref_axis',(1.41426179436738E-51,-1.,-5.60383084497445E-34)) ;
#62756=DIRECTION('',(0.,0.,-1.)) ;
#62757=DIRECTION('',(1.41426179436738E-51,-1.,-5.60383084497445E-34)) ;
#62758=DIRECTION('center_axis',(0.,-1.,0.)) ;
#62759=DIRECTION('ref_axis',(-1.,0.,-2.52374105052742E-18)) ;
#62760=DIRECTION('',(0.,0.,-1.)) ;
#62761=DIRECTION('',(-1.,0.,-2.52374105052742E-18)) ;
#62762=DIRECTION('center_axis',(-1.,-1.41426179436738E-51,0.)) ;
#62763=DIRECTION('ref_axis',(-1.41426179436738E-51,1.,5.60383084497445E-34)) ;
#62764=DIRECTION('',(0.,0.,-1.)) ;
#62765=DIRECTION('',(-1.41426179436738E-51,1.,5.60383084497445E-34)) ;
#62766=DIRECTION('center_axis',(0.,-1.,0.)) ;
#62767=DIRECTION('ref_axis',(-1.,0.,-2.52374105052742E-18)) ;
#62768=DIRECTION('',(0.,0.,-1.)) ;
#62769=DIRECTION('',(-1.,0.,-2.52374105052742E-18)) ;
#62770=DIRECTION('center_axis',(0.,0.,-1.)) ;
#62771=DIRECTION('ref_axis',(-1.,0.,0.)) ;
#62772=DIRECTION('center_axis',(2.52374105052742E-18,5.60383084497445E-34,
-1.)) ;
#62773=DIRECTION('ref_axis',(-1.,0.,0.)) ;
#62774=DIRECTION('center_axis',(-2.52374105052742E-18,-5.60383084497445E-34,
1.)) ;
#62775=DIRECTION('ref_axis',(1.,-2.24153233798973E-35,2.52374105052742E-18)) ;
#62776=DIRECTION('center_axis',(0.,-1.,-5.60383084497445E-34)) ;
#62777=DIRECTION('ref_axis',(1.,0.,0.)) ;
#62778=DIRECTION('center_axis',(2.52374105052742E-18,5.60383084497445E-34,
-1.)) ;
#62779=DIRECTION('ref_axis',(1.,-2.24153233798973E-35,2.52374105052742E-18)) ;
#62780=DIRECTION('center_axis',(2.52374105052742E-18,5.60383084497445E-34,
-1.)) ;
#62781=DIRECTION('ref_axis',(1.,-2.24153233798973E-35,2.52374105052742E-18)) ;
#62782=DIRECTION('center_axis',(0.,0.,-1.)) ;
#62783=DIRECTION('ref_axis',(1.,0.,0.)) ;
#62784=DIRECTION('',(0.,0.,1.)) ;
#62785=DIRECTION('center_axis',(-2.52374105052742E-18,-5.60383084497445E-34,
1.)) ;
#62786=DIRECTION('ref_axis',(1.,4.48306467597956E-35,2.52374105052742E-18)) ;
#62787=DIRECTION('center_axis',(-2.52374105052742E-18,-5.60383084497445E-34,
1.)) ;
#62788=DIRECTION('ref_axis',(1.,4.48306467597956E-35,2.52374105052742E-18)) ;
#62789=DIRECTION('center_axis',(2.52374105052742E-18,5.60383084497445E-34,
-1.)) ;
#62790=DIRECTION('ref_axis',(1.,3.40207761657885E-68,2.52374105052742E-18)) ;
#62791=DIRECTION('center_axis',(-1.,0.,-2.52374105052742E-18)) ;
#62792=DIRECTION('ref_axis',(-1.78455441078696E-18,0.707106781186485,0.70710678118661)) ;
#62793=DIRECTION('',(1.,0.,2.52374105052742E-18)) ;
#62794=DIRECTION('center_axis',(-0.70710678118661,-0.707106781186485,0.)) ;
#62795=DIRECTION('ref_axis',(0.707106781186485,-0.70710678118661,3.56910882157392E-18)) ;
#62796=DIRECTION('center_axis',(-0.70710678118661,0.707106781186485,0.)) ;
#62797=DIRECTION('ref_axis',(-0.707106781186485,-0.70710678118661,-7.92501358220685E-34)) ;
#62798=DIRECTION('center_axis',(1.41426179436738E-51,-1.,-5.60383084497445E-34)) ;
#62799=DIRECTION('ref_axis',(-0.707106781186548,-3.96250679110377E-34,0.707106781186548)) ;
#62800=DIRECTION('',(-1.41426179436738E-51,1.,5.60383084497445E-34)) ;
#62801=DIRECTION('center_axis',(-0.70710678118661,-0.707106781186485,0.)) ;
#62802=DIRECTION('ref_axis',(-0.707106781186485,0.70710678118661,7.92501358220685E-34)) ;
#62803=DIRECTION('center_axis',(-1.,0.,-2.52374105052742E-18)) ;
#62804=DIRECTION('ref_axis',(-1.78455441078696E-18,0.707106781186485,0.70710678118661)) ;
#62805=DIRECTION('',(1.,0.,2.52374105052742E-18)) ;
#62806=DIRECTION('center_axis',(-0.70710678118661,-0.707106781186485,0.)) ;
#62807=DIRECTION('ref_axis',(0.707106781186485,-0.70710678118661,3.56910882157392E-18)) ;
#62808=DIRECTION('center_axis',(1.41426179436738E-51,-1.,-5.60383084497445E-34)) ;
#62809=DIRECTION('ref_axis',(-0.707106781186548,-3.96250679110377E-34,0.707106781186548)) ;
#62810=DIRECTION('',(-1.41426179436738E-51,1.,5.60383084497445E-34)) ;
#62811=DIRECTION('center_axis',(0.70710678118661,-0.707106781186485,0.)) ;
#62812=DIRECTION('ref_axis',(0.707106781186485,0.70710678118661,7.92501358220685E-34)) ;
#62813=DIRECTION('center_axis',(1.,0.,2.52374105052742E-18)) ;
#62814=DIRECTION('ref_axis',(-1.78455441078696E-18,-0.707106781186485,0.70710678118661)) ;
#62815=DIRECTION('',(-1.,0.,-2.52374105052742E-18)) ;
#62816=DIRECTION('center_axis',(0.70710678118661,-0.707106781186485,0.)) ;
#62817=DIRECTION('ref_axis',(-0.707106781186485,-0.70710678118661,-3.56910882157392E-18)) ;
#62818=DIRECTION('',(1.,0.,2.52374105052742E-18)) ;
#62819=DIRECTION('center_axis',(1.,0.,2.52374105052742E-18)) ;
#62820=DIRECTION('ref_axis',(-1.78455441078696E-18,-0.707106781186485,0.70710678118661)) ;
#62821=DIRECTION('',(-1.,0.,-2.52374105052742E-18)) ;
#62822=DIRECTION('center_axis',(0.70710678118661,0.707106781186485,0.)) ;
#62823=DIRECTION('ref_axis',(-0.707106781186485,0.70710678118661,-3.56910882157392E-18)) ;
#62824=DIRECTION('',(1.,0.,2.52374105052742E-18)) ;
#62825=DIRECTION('center_axis',(-0.70710678118661,0.707106781186485,0.)) ;
#62826=DIRECTION('ref_axis',(-0.707106781186485,-0.70710678118661,-3.56910882157392E-18)) ;
#62827=DIRECTION('center_axis',(-1.41426179436738E-51,1.,5.60383084497445E-34)) ;
#62828=DIRECTION('ref_axis',(0.707106781186548,-3.96250679110377E-34,0.707106781186548)) ;
#62829=DIRECTION('',(-1.41426179436738E-51,1.,5.60383084497445E-34)) ;
#62830=DIRECTION('',(1.41426179436738E-51,-1.,-5.60383084497445E-34)) ;
#62831=DIRECTION('center_axis',(0.70710678118661,0.707106781186485,0.)) ;
#62832=DIRECTION('ref_axis',(0.707106781186485,-0.70710678118661,-7.92501358220685E-34)) ;
#62833=DIRECTION('center_axis',(1.41426179436738E-51,-1.,-5.60383084497445E-34)) ;
#62834=DIRECTION('ref_axis',(-0.707106781186548,-3.96250679110377E-34,0.707106781186548)) ;
#62835=DIRECTION('',(-1.41426179436738E-51,1.,5.60383084497445E-34)) ;
#62836=DIRECTION('',(1.41426179436738E-51,-1.,-5.60383084497445E-34)) ;
#62837=DIRECTION('center_axis',(1.,0.,2.52374105052742E-18)) ;
#62838=DIRECTION('ref_axis',(-1.78455441078696E-18,-0.707106781186485,0.70710678118661)) ;
#62839=DIRECTION('',(1.,0.,2.52374105052742E-18)) ;
#62840=DIRECTION('',(-1.,0.,-2.52374105052742E-18)) ;
#62841=DIRECTION('center_axis',(0.70710678118661,0.707106781186485,0.)) ;
#62842=DIRECTION('ref_axis',(-0.707106781186485,0.70710678118661,-3.56910882157392E-18)) ;
#62843=DIRECTION('center_axis',(-1.41426179436738E-51,1.,5.60383084497445E-34)) ;
#62844=DIRECTION('ref_axis',(0.707106781186548,-3.96250679110377E-34,0.707106781186548)) ;
#62845=DIRECTION('',(-1.41426179436738E-51,1.,5.60383084497445E-34)) ;
#62846=DIRECTION('',(1.41426179436738E-51,-1.,-5.60383084497445E-34)) ;
#62847=DIRECTION('center_axis',(-0.70710678118661,0.707106781186485,0.)) ;
#62848=DIRECTION('ref_axis',(-0.707106781186485,-0.70710678118661,-7.92501358220685E-34)) ;
#62849=DIRECTION('center_axis',(-1.,0.,-2.52374105052742E-18)) ;
#62850=DIRECTION('ref_axis',(-1.78455441078696E-18,0.707106781186485,0.70710678118661)) ;
#62851=DIRECTION('',(1.,0.,2.52374105052742E-18)) ;
#62852=DIRECTION('center_axis',(-0.70710678118661,0.707106781186485,0.)) ;
#62853=DIRECTION('ref_axis',(0.707106781186485,0.70710678118661,3.56910882157392E-18)) ;
#62854=DIRECTION('center_axis',(-1.41426179436738E-51,1.,5.60383084497445E-34)) ;
#62855=DIRECTION('ref_axis',(0.707106781186548,-3.96250679110377E-34,0.707106781186548)) ;
#62856=DIRECTION('',(1.41426179436738E-51,-1.,-5.60383084497445E-34)) ;
#62857=DIRECTION('center_axis',(0.,1.,0.)) ;
#62858=DIRECTION('ref_axis',(1.,0.,2.52374105052742E-18)) ;
#62859=DIRECTION('',(0.,0.,-1.)) ;
#62860=DIRECTION('center_axis',(1.,1.41426179436738E-51,0.)) ;
#62861=DIRECTION('ref_axis',(1.41426179436738E-51,-1.,-5.60383084497445E-34)) ;
#62862=DIRECTION('',(0.,0.,-1.)) ;
#62863=DIRECTION('center_axis',(0.,1.,0.)) ;
#62864=DIRECTION('ref_axis',(1.,0.,2.52374105052742E-18)) ;
#62865=DIRECTION('',(0.,0.,-1.)) ;
#62866=DIRECTION('center_axis',(2.52374105052742E-18,5.60383084497445E-34,
-1.)) ;
#62867=DIRECTION('ref_axis',(1.,3.40207761657885E-68,2.52374105052742E-18)) ;
#62868=DIRECTION('center_axis',(2.52374105052742E-18,5.60383084497445E-34,
-1.)) ;
#62869=DIRECTION('ref_axis',(1.,4.48306467597956E-35,2.52374105052742E-18)) ;
#62870=DIRECTION('center_axis',(2.52374105052742E-18,5.60383084497445E-34,
-1.)) ;
#62871=DIRECTION('ref_axis',(-1.,0.,0.)) ;
#62872=DIRECTION('center_axis',(0.,-1.,-5.60383084497445E-34)) ;
#62873=DIRECTION('ref_axis',(1.,0.,0.)) ;
#62874=DIRECTION('center_axis',(-1.,-1.41426179436738E-51,0.)) ;
#62875=DIRECTION('ref_axis',(-1.41426179436738E-51,1.,5.60383084497445E-34)) ;
#62876=DIRECTION('',(0.,0.,-1.)) ;
#62877=DIRECTION('center_axis',(0.,1.,0.)) ;
#62878=DIRECTION('ref_axis',(1.,0.,2.52374105052742E-18)) ;
#62879=DIRECTION('',(0.,0.,-1.)) ;
#62880=DIRECTION('center_axis',(-1.,-1.41426179436738E-51,0.)) ;
#62881=DIRECTION('ref_axis',(-1.41426179436738E-51,1.,5.60383084497445E-34)) ;
#88582=CARTESIAN_POINT('',(0.,0.,0.)) ;
#88583=CARTESIAN_POINT('Origin',(30.55,254.6,30.0213203435596)) ;
#88584=CARTESIAN_POINT('',(30.5,254.6,29.9213203435596)) ;
#88585=CARTESIAN_POINT('',(29.3,254.6,29.9213203435596)) ;
#88586=CARTESIAN_POINT('',(30.55,254.6,29.9213203435596)) ;
#88587=CARTESIAN_POINT('',(29.2,254.5,30.0213203435596)) ;
#88588=CARTESIAN_POINT('Origin',(29.3,254.6,30.0213203435596)) ;
#88589=CARTESIAN_POINT('',(30.4,254.5,30.0213203435596)) ;
#88590=CARTESIAN_POINT('',(30.55,254.5,30.0213203435596)) ;
#88591=CARTESIAN_POINT('Origin',(30.5,254.6,30.0213203435596)) ;
#88592=CARTESIAN_POINT('Origin',(29.3,254.65,30.0213203435596)) ;
#88593=CARTESIAN_POINT('',(29.3,255.,29.9213203435596)) ;
#88594=CARTESIAN_POINT('',(29.3,254.65,29.9213203435596)) ;
#88595=CARTESIAN_POINT('',(29.2,255.1,30.0213203435596)) ;
#88596=CARTESIAN_POINT('Origin',(29.3,255.,30.0213203435596)) ;
#88597=CARTESIAN_POINT('',(29.2,254.65,30.0213203435596)) ;
#88598=CARTESIAN_POINT('Origin',(29.95,255.,30.0213203435596)) ;
#88599=CARTESIAN_POINT('',(30.5,255.,29.9213203435596)) ;
#88600=CARTESIAN_POINT('',(29.95,255.,29.9213203435596)) ;
#88601=CARTESIAN_POINT('',(30.4,255.1,30.0213203435596)) ;
#88602=CARTESIAN_POINT('Origin',(30.5,255.,30.0213203435596)) ;
#88603=CARTESIAN_POINT('',(29.95,255.1,30.0213203435596)) ;
#88604=CARTESIAN_POINT('Origin',(30.5,254.95,30.0213203435596)) ;
#88605=CARTESIAN_POINT('',(30.5,256.2,29.9213203435596)) ;
#88606=CARTESIAN_POINT('',(30.5,254.95,29.9213203435596)) ;
#88607=CARTESIAN_POINT('',(30.4,256.3,30.0213203435596)) ;
#88608=CARTESIAN_POINT('Origin',(30.5,256.2,30.0213203435596)) ;
#88609=CARTESIAN_POINT('',(30.4,254.95,30.0213203435596)) ;
#88610=CARTESIAN_POINT('Origin',(30.55,256.2,30.0213203435596)) ;
#88611=CARTESIAN_POINT('',(30.9,256.2,29.9213203435596)) ;
#88612=CARTESIAN_POINT('',(30.55,256.2,29.9213203435596)) ;
#88613=CARTESIAN_POINT('',(31.,256.3,30.0213203435596)) ;
#88614=CARTESIAN_POINT('Origin',(30.9,256.2,30.0213203435596)) ;
#88615=CARTESIAN_POINT('',(30.55,256.3,30.0213203435596)) ;
#88616=CARTESIAN_POINT('Origin',(30.9,255.55,30.0213203435596)) ;
#88617=CARTESIAN_POINT('',(31.,255.1,30.0213203435596)) ;
#88618=CARTESIAN_POINT('',(31.,255.55,30.0213203435596)) ;
#88619=CARTESIAN_POINT('',(30.9,255.,29.9213203435596)) ;
#88620=CARTESIAN_POINT('',(30.9,255.55,29.9213203435596)) ;
#88621=CARTESIAN_POINT('Origin',(30.9,255.,30.0213203435596)) ;
#88622=CARTESIAN_POINT('Origin',(30.85,255.,30.0213203435596)) ;
#88623=CARTESIAN_POINT('',(32.2,255.1,30.0213203435596)) ;
#88624=CARTESIAN_POINT('',(30.85,255.1,30.0213203435596)) ;
#88625=CARTESIAN_POINT('',(32.1,255.,29.9213203435596)) ;
#88626=CARTESIAN_POINT('',(30.85,255.,29.9213203435596)) ;
#88627=CARTESIAN_POINT('Origin',(32.1,255.,30.0213203435596)) ;
#88628=CARTESIAN_POINT('Origin',(32.1,254.95,30.0213203435596)) ;
#88629=CARTESIAN_POINT('',(32.2,254.5,30.0213203435596)) ;
#88630=CARTESIAN_POINT('',(32.2,254.95,30.0213203435596)) ;
#88631=CARTESIAN_POINT('',(32.1,254.6,29.9213203435596)) ;
#88632=CARTESIAN_POINT('',(32.1,254.95,29.9213203435596)) ;
#88633=CARTESIAN_POINT('Origin',(32.1,254.6,30.0213203435596)) ;
#88634=CARTESIAN_POINT('Origin',(31.45,254.6,30.0213203435596)) ;
#88635=CARTESIAN_POINT('',(31.,254.5,30.0213203435596)) ;
#88636=CARTESIAN_POINT('',(31.45,254.5,30.0213203435596)) ;
#88637=CARTESIAN_POINT('',(30.9,254.6,29.9213203435596)) ;
#88638=CARTESIAN_POINT('',(31.45,254.6,29.9213203435596)) ;
#88639=CARTESIAN_POINT('Origin',(30.9,254.6,30.0213203435596)) ;
#88640=CARTESIAN_POINT('Origin',(30.9,254.65,30.0213203435596)) ;
#88641=CARTESIAN_POINT('',(31.,253.3,30.0213203435596)) ;
#88642=CARTESIAN_POINT('',(31.,254.65,30.0213203435596)) ;
#88643=CARTESIAN_POINT('',(30.9,253.4,29.9213203435596)) ;
#88644=CARTESIAN_POINT('',(30.9,254.65,29.9213203435596)) ;
#88645=CARTESIAN_POINT('Origin',(30.9,253.4,30.0213203435596)) ;
#88646=CARTESIAN_POINT('Origin',(30.85,253.4,30.0213203435596)) ;
#88647=CARTESIAN_POINT('',(30.4,253.3,30.0213203435596)) ;
#88648=CARTESIAN_POINT('',(30.85,253.3,30.0213203435596)) ;
#88649=CARTESIAN_POINT('',(30.5,253.4,29.9213203435596)) ;
#88650=CARTESIAN_POINT('',(30.85,253.4,29.9213203435596)) ;
#88651=CARTESIAN_POINT('Origin',(30.5,253.4,30.0213203435596)) ;
#88652=CARTESIAN_POINT('Origin',(30.5,254.05,30.0213203435596)) ;
#88653=CARTESIAN_POINT('',(30.4,254.05,30.0213203435596)) ;
#88654=CARTESIAN_POINT('',(30.5,254.05,29.9213203435596)) ;
#88655=CARTESIAN_POINT('Origin',(32.2,255.1,30.7213203435596)) ;
#88656=CARTESIAN_POINT('',(32.2,254.5,30.1213203435596)) ;
#88657=CARTESIAN_POINT('',(32.2,254.5,30.7213203435596)) ;
#88658=CARTESIAN_POINT('',(32.2,255.1,30.1213203435596)) ;
#88659=CARTESIAN_POINT('',(32.2,254.95,30.1213203435596)) ;
#88660=CARTESIAN_POINT('',(32.2,255.1,30.7213203435596)) ;
#88661=CARTESIAN_POINT('Origin',(32.2,254.5,30.7213203435596)) ;
#88662=CARTESIAN_POINT('',(31.,254.5,30.1213203435596)) ;
#88663=CARTESIAN_POINT('',(31.,254.5,30.7213203435596)) ;
#88664=CARTESIAN_POINT('',(31.45,254.5,30.1213203435596)) ;
#88665=CARTESIAN_POINT('Origin',(31.,254.5,30.7213203435596)) ;
#88666=CARTESIAN_POINT('',(31.,253.3,30.1213203435596)) ;
#88667=CARTESIAN_POINT('',(31.,253.3,30.7213203435596)) ;
#88668=CARTESIAN_POINT('',(31.,254.65,30.1213203435596)) ;
#88669=CARTESIAN_POINT('Origin',(31.,253.3,30.7213203435596)) ;
#88670=CARTESIAN_POINT('',(30.4,253.3,30.1213203435596)) ;
#88671=CARTESIAN_POINT('',(30.4,253.3,30.7213203435596)) ;
#88672=CARTESIAN_POINT('',(30.85,253.3,30.1213203435596)) ;
#88673=CARTESIAN_POINT('Origin',(30.4,253.3,30.7213203435596)) ;
#88674=CARTESIAN_POINT('',(30.4,254.5,30.1213203435596)) ;
#88675=CARTESIAN_POINT('',(30.4,254.5,30.7213203435596)) ;
#88676=CARTESIAN_POINT('',(30.4,254.05,30.1213203435596)) ;
#88677=CARTESIAN_POINT('Origin',(30.4,254.5,30.7213203435596)) ;
#88678=CARTESIAN_POINT('',(29.2,254.5,30.1213203435596)) ;
#88679=CARTESIAN_POINT('',(29.2,254.5,30.7213203435596)) ;
#88680=CARTESIAN_POINT('',(30.55,254.5,30.1213203435596)) ;
#88681=CARTESIAN_POINT('Origin',(30.7,254.8,29.9213203435596)) ;
#88682=CARTESIAN_POINT('Origin',(30.7,254.8,28.8213203435596)) ;
#88683=CARTESIAN_POINT('',(33.1,254.8,28.7213203435596)) ;
#88684=CARTESIAN_POINT('Origin',(30.7,254.8,28.7213203435596)) ;
#88685=CARTESIAN_POINT('',(33.2,254.8,28.8213203435596)) ;
#88686=CARTESIAN_POINT('Origin',(33.1,254.8,28.8213203435596)) ;
#88687=CARTESIAN_POINT('',(28.2,254.8,28.8213203435596)) ;
#88688=CARTESIAN_POINT('Origin',(30.7,254.8,28.8213203435596)) ;
#88689=CARTESIAN_POINT('Origin',(30.7,254.8,28.8213203435596)) ;
#88690=CARTESIAN_POINT('Origin',(30.7,254.8,30.2213203435596)) ;
#88691=CARTESIAN_POINT('',(28.2,254.8,30.0213203435596)) ;
#88692=CARTESIAN_POINT('',(28.2,254.8,30.2213203435596)) ;
#88693=CARTESIAN_POINT('',(33.2,254.8,30.0213203435596)) ;
#88694=CARTESIAN_POINT('Origin',(30.7,254.8,30.0213203435596)) ;
#88695=CARTESIAN_POINT('Origin',(30.7,254.8,30.0213203435596)) ;
#88696=CARTESIAN_POINT('Origin',(30.7,254.8,28.7213203435596)) ;
#88697=CARTESIAN_POINT('Origin',(30.85,253.2,30.1213203435596)) ;
#88698=CARTESIAN_POINT('',(30.3,253.2,30.2213203435596)) ;
#88699=CARTESIAN_POINT('',(31.1,253.2,30.2213203435596)) ;
#88700=CARTESIAN_POINT('',(30.85,253.2,30.2213203435596)) ;
#88701=CARTESIAN_POINT('Origin',(31.1,253.2,30.1213203435596)) ;
#88702=CARTESIAN_POINT('Origin',(30.3,253.2,30.1213203435596)) ;
#88703=CARTESIAN_POINT('Origin',(31.1,254.65,30.1213203435596)) ;
#88704=CARTESIAN_POINT('',(31.1,254.4,30.2213203435596)) ;
#88705=CARTESIAN_POINT('',(31.1,254.65,30.2213203435596)) ;
#88706=CARTESIAN_POINT('Origin',(31.1,254.4,30.1213203435596)) ;
#88707=CARTESIAN_POINT('Origin',(31.45,254.4,30.1213203435596)) ;
#88708=CARTESIAN_POINT('',(32.3,254.4,30.2213203435596)) ;
#88709=CARTESIAN_POINT('',(31.45,254.4,30.2213203435596)) ;
#88710=CARTESIAN_POINT('Origin',(32.3,254.4,30.1213203435596)) ;
#88711=CARTESIAN_POINT('Origin',(32.3,254.95,30.1213203435596)) ;
#88712=CARTESIAN_POINT('',(32.3,255.2,30.2213203435596)) ;
#88713=CARTESIAN_POINT('',(32.3,254.95,30.2213203435596)) ;
#88714=CARTESIAN_POINT('Origin',(32.3,255.2,30.1213203435596)) ;
#88715=CARTESIAN_POINT('Origin',(30.85,255.2,30.1213203435596)) ;
#88716=CARTESIAN_POINT('',(31.1,255.2,30.2213203435596)) ;
#88717=CARTESIAN_POINT('',(30.85,255.2,30.2213203435596)) ;
#88718=CARTESIAN_POINT('',(31.,255.1,30.1213203435596)) ;
#88719=CARTESIAN_POINT('Origin',(31.1,255.2,30.1213203435596)) ;
#88720=CARTESIAN_POINT('',(30.85,255.1,30.1213203435596)) ;
#88721=CARTESIAN_POINT('Origin',(30.55,256.4,30.1213203435596)) ;
#88722=CARTESIAN_POINT('',(31.1,256.4,30.2213203435596)) ;
#88723=CARTESIAN_POINT('',(30.3,256.4,30.2213203435596)) ;
#88724=CARTESIAN_POINT('',(30.55,256.4,30.2213203435596)) ;
#88725=CARTESIAN_POINT('',(30.4,256.3,30.1213203435596)) ;
#88726=CARTESIAN_POINT('Origin',(30.3,256.4,30.1213203435596)) ;
#88727=CARTESIAN_POINT('',(31.,256.3,30.1213203435596)) ;
#88728=CARTESIAN_POINT('',(30.55,256.3,30.1213203435596)) ;
#88729=CARTESIAN_POINT('Origin',(31.1,256.4,30.1213203435596)) ;
#88730=CARTESIAN_POINT('Origin',(30.3,254.95,30.1213203435596)) ;
#88731=CARTESIAN_POINT('',(30.4,255.1,30.1213203435596)) ;
#88732=CARTESIAN_POINT('',(30.4,254.95,30.1213203435596)) ;
#88733=CARTESIAN_POINT('',(30.3,255.2,30.2213203435596)) ;
#88734=CARTESIAN_POINT('',(30.3,254.95,30.2213203435596)) ;
#88735=CARTESIAN_POINT('Origin',(30.3,255.2,30.1213203435596)) ;
#88736=CARTESIAN_POINT('Origin',(31.1,255.55,30.1213203435596)) ;
#88737=CARTESIAN_POINT('',(31.1,255.55,30.2213203435596)) ;
#88738=CARTESIAN_POINT('',(31.,255.55,30.1213203435596)) ;
#88739=CARTESIAN_POINT('Origin',(29.95,255.2,30.1213203435596)) ;
#88740=CARTESIAN_POINT('',(29.2,255.1,30.1213203435596)) ;
#88741=CARTESIAN_POINT('',(29.95,255.1,30.1213203435596)) ;
#88742=CARTESIAN_POINT('',(29.1,255.2,30.2213203435596)) ;
#88743=CARTESIAN_POINT('',(29.95,255.2,30.2213203435596)) ;
#88744=CARTESIAN_POINT('Origin',(29.1,255.2,30.1213203435596)) ;
#88745=CARTESIAN_POINT('Origin',(29.1,254.65,30.1213203435596)) ;
#88746=CARTESIAN_POINT('',(29.2,254.65,30.1213203435596)) ;
#88747=CARTESIAN_POINT('',(29.1,254.4,30.2213203435596)) ;
#88748=CARTESIAN_POINT('',(29.1,254.65,30.2213203435596)) ;
#88749=CARTESIAN_POINT('Origin',(29.1,254.4,30.1213203435596)) ;
#88750=CARTESIAN_POINT('Origin',(30.55,254.4,30.1213203435596)) ;
#88751=CARTESIAN_POINT('',(30.3,254.4,30.2213203435596)) ;
#88752=CARTESIAN_POINT('',(30.55,254.4,30.2213203435596)) ;
#88753=CARTESIAN_POINT('Origin',(30.3,254.4,30.1213203435596)) ;
#88754=CARTESIAN_POINT('Origin',(30.3,254.05,30.1213203435596)) ;
#88755=CARTESIAN_POINT('',(30.3,254.05,30.2213203435596)) ;
#88756=CARTESIAN_POINT('Origin',(31.,255.1,30.7213203435596)) ;
#88757=CARTESIAN_POINT('',(31.,255.1,30.7213203435596)) ;
#88758=CARTESIAN_POINT('Origin',(31.,256.3,30.7213203435596)) ;
#88759=CARTESIAN_POINT('',(31.,256.3,30.7213203435596)) ;
#88760=CARTESIAN_POINT('Origin',(30.4,256.3,30.7213203435596)) ;
#88761=CARTESIAN_POINT('',(30.4,256.3,30.7213203435596)) ;
#88762=CARTESIAN_POINT('Origin',(30.7,254.8,30.2213203435596)) ;
#88763=CARTESIAN_POINT('',(33.,254.8,30.2213203435596)) ;
#88764=CARTESIAN_POINT('Origin',(30.7,254.8,30.2213203435596)) ;
#88765=CARTESIAN_POINT('Origin',(30.7,254.8,30.0213203435596)) ;
#88766=CARTESIAN_POINT('Origin',(33.,254.8,30.0213203435596)) ;
#88767=CARTESIAN_POINT('Origin',(29.2,254.5,30.7213203435596)) ;
#88768=CARTESIAN_POINT('',(29.2,255.1,30.7213203435596)) ;
#88769=CARTESIAN_POINT('Origin',(29.2,255.1,30.7213203435596)) ;
#88770=CARTESIAN_POINT('',(30.4,255.1,30.7213203435596)) ;
#88771=CARTESIAN_POINT('Origin',(30.4,255.1,30.7213203435596)) ;
#117139=UNCERTAINTY_MEASURE_WITH_UNIT(LENGTH_MEASURE(0.01),#117171,
'DISTANCE_ACCURACY_VALUE',
'Maximum model space distance between geometric entities at asserted c
onnectivities') ;
#117147=UNCERTAINTY_MEASURE_WITH_UNIT(LENGTH_MEASURE(0.01),#117171,
'DISTANCE_ACCURACY_VALUE',
'Maximum model space distance between geometric entities at asserted c
onnectivities') ;
#117162=(
GEOMETRIC_REPRESENTATION_CONTEXT(3)
GLOBAL_UNCERTAINTY_ASSIGNED_CONTEXT((#117139))
GLOBAL_UNIT_ASSIGNED_CONTEXT((#117171,#117173,#117174))
REPRESENTATION_CONTEXT('','3D')
) ;
#117170=(
GEOMETRIC_REPRESENTATION_CONTEXT(3)
GLOBAL_UNCERTAINTY_ASSIGNED_CONTEXT((#117147))
GLOBAL_UNIT_ASSIGNED_CONTEXT((#117171,#117173,#117174))
REPRESENTATION_CONTEXT('','3D')
) ;
#117171=(
LENGTH_UNIT()
NAMED_UNIT(*)
SI_UNIT(.MILLI.,.METRE.)
) ;
#117173=(
NAMED_UNIT(*)
PLANE_ANGLE_UNIT()
SI_UNIT($,.RADIAN.)
) ;
#117174=(
NAMED_UNIT(*)
SI_UNIT($,.STERADIAN.)
SOLID_ANGLE_UNIT()
) ;
#117189=SHAPE_DEFINITION_REPRESENTATION(#117211,#117254) ;
#117211=PRODUCT_DEFINITION_SHAPE('',$,#117277) ;
#117254=SHAPE_REPRESENTATION('',(#52369),#117162) ;
#117262=PRODUCT_DEFINITION_CONTEXT('part definition',#117330,'design') ;
#117277=PRODUCT_DEFINITION('Spacer_3','Spacer_3',#117299,#117262) ;
#117299=PRODUCT_DEFINITION_FORMATION('',$,#117346) ;
#117330=APPLICATION_CONTEXT(
'Core Data for Automotive Mechanical Design Process') ;
#117331=PRODUCT_CONTEXT('part definition',#117330,'mechanical') ;
#117346=PRODUCT('Spacer_3','Spacer_3',$,(#117331)) ;
#117355=PRESENTATION_STYLE_ASSIGNMENT((#117357)) ;
#117357=SURFACE_STYLE_USAGE(.BOTH.,#117359) ;
#117359=SURFACE_SIDE_STYLE('',(#117361)) ;
#117361=SURFACE_STYLE_FILL_AREA(#117363) ;
#117363=FILL_AREA_STYLE('Opaque(160,160,160)',(#117365)) ;
#117365=FILL_AREA_STYLE_COLOUR('Opaque(160,160,160)',#117367) ;
#117367=COLOUR_RGB('Opaque(160,160,160)', 0.09019608, 0.27058824, 0.51372549) ;
ENDSEC;
END-ISO-10303-21;
